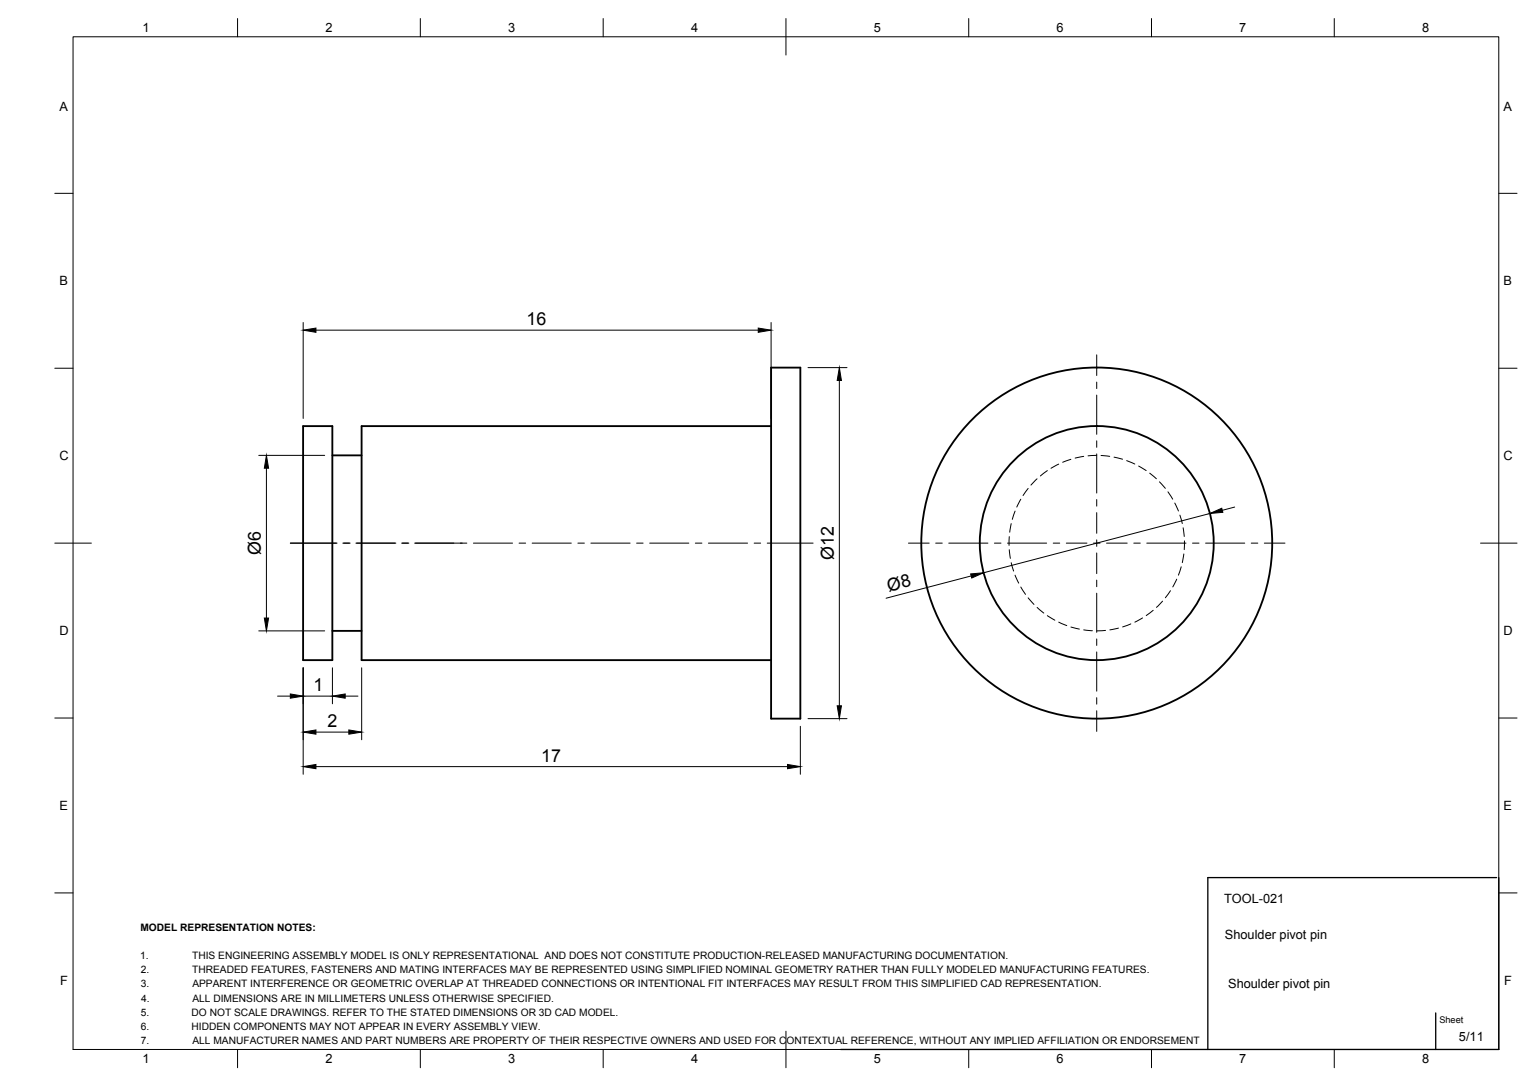
ISO-10303-21;
HEADER;
/* Generated by software containing ST-Developer
 * from STEP Tools, Inc. (www.steptools.com) 
 */

FILE_DESCRIPTION(
/* description */ (''),
/* implementation_level */ '2;1');

FILE_NAME(
/* name */ 'Shoulder pivot pin.step',
/* time_stamp */ '2026-11-10T09:05:57-08:00',
/* author */ (''),
/* organization */ (''),
/* preprocessor_version */ 'ST-DEVELOPER v20.2',
/* originating_system */ 'Autodesk Translation Framework v15.17.0.0',
/* authorisation */ '');

FILE_SCHEMA (('AUTOMOTIVE_DESIGN { 1 0 10303 214 3 1 1 }'));
ENDSEC;

DATA;
#10=MECHANICAL_DESIGN_GEOMETRIC_PRESENTATION_REPRESENTATION('',(#567),#19618);
#547=SHAPE_REPRESENTATION_RELATIONSHIP('SRR','None',#19666,#557);
#557=ADVANCED_BREP_SHAPE_REPRESENTATION('',(#577),#19609);
#567=STYLED_ITEM('',(#19729),#577);
#577=MANIFOLD_SOLID_BREP('Body1',#7105);
#605=FACE_BOUND('',#1304,.T.);
#606=FACE_BOUND('',#1306,.T.);
#607=FACE_BOUND('',#1309,.T.);
#698=PLANE('',#7347);
#699=PLANE('',#7349);
#700=PLANE('',#7353);
#701=PLANE('',#7358);
#702=PLANE('',#7360);
#883=FACE_OUTER_BOUND('',#1302,.T.);
#884=FACE_OUTER_BOUND('',#1303,.T.);
#885=FACE_OUTER_BOUND('',#1305,.T.);
#886=FACE_OUTER_BOUND('',#1307,.T.);
#887=FACE_OUTER_BOUND('',#1308,.T.);
#888=FACE_OUTER_BOUND('',#1310,.T.);
#889=FACE_OUTER_BOUND('',#1311,.T.);
#890=FACE_OUTER_BOUND('',#1312,.T.);
#891=FACE_OUTER_BOUND('',#1313,.T.);
#1302=EDGE_LOOP('',(#4842,#4843,#4844,#4845));
#1303=EDGE_LOOP('',(#4846));
#1304=EDGE_LOOP('',(#4847));
#1305=EDGE_LOOP('',(#4848));
#1306=EDGE_LOOP('',(#4849));
#1307=EDGE_LOOP('',(#4850,#4851,#4852,#4853));
#1308=EDGE_LOOP('',(#4854));
#1309=EDGE_LOOP('',(#4855));
#1310=EDGE_LOOP('',(#4856,#4857,#4858,#4859));
#1311=EDGE_LOOP('',(#4860));
#1312=EDGE_LOOP('',(#4861,#4862,#4863,#4864));
#1313=EDGE_LOOP('',(#4865));
#1813=LINE('',#9668,#2272);
#1814=LINE('',#9679,#2273);
#1815=LINE('',#9687,#2274);
#1816=LINE('',#9691,#2275);
#2272=VECTOR('',#8128,0.3);
#2273=VECTOR('',#8143,0.4);
#2274=VECTOR('',#8152,0.6);
#2275=VECTOR('',#8159,0.4);
#2670=CIRCLE('',#7345,0.3);
#2671=CIRCLE('',#7346,0.3);
#2672=CIRCLE('',#7348,0.4);
#2673=CIRCLE('',#7350,0.4);
#2674=CIRCLE('',#7352,0.4);
#2675=CIRCLE('',#7354,0.6);
#2676=CIRCLE('',#7355,0.4);
#2677=CIRCLE('',#7357,0.6);
#2921=VERTEX_POINT('',#9665);
#2922=VERTEX_POINT('',#9667);
#2923=VERTEX_POINT('',#9671);
#2924=VERTEX_POINT('',#9674);
#2925=VERTEX_POINT('',#9677);
#2926=VERTEX_POINT('',#9681);
#2927=VERTEX_POINT('',#9683);
#2928=VERTEX_POINT('',#9686);
#3646=EDGE_CURVE('',#2921,#2921,#2670,.T.);
#3647=EDGE_CURVE('',#2921,#2922,#1813,.T.);
#3648=EDGE_CURVE('',#2922,#2922,#2671,.T.);
#3649=EDGE_CURVE('',#2923,#2923,#2672,.T.);
#3650=EDGE_CURVE('',#2924,#2924,#2673,.T.);
#3651=EDGE_CURVE('',#2925,#2925,#2674,.T.);
#3652=EDGE_CURVE('',#2925,#2924,#1814,.T.);
#3653=EDGE_CURVE('',#2926,#2926,#2675,.T.);
#3654=EDGE_CURVE('',#2927,#2927,#2676,.T.);
#3655=EDGE_CURVE('',#2926,#2928,#1815,.T.);
#3656=EDGE_CURVE('',#2928,#2928,#2677,.T.);
#3657=EDGE_CURVE('',#2923,#2927,#1816,.T.);
#4842=ORIENTED_EDGE('',*,*,#3646,.T.);
#4843=ORIENTED_EDGE('',*,*,#3647,.T.);
#4844=ORIENTED_EDGE('',*,*,#3648,.F.);
#4845=ORIENTED_EDGE('',*,*,#3647,.F.);
#4846=ORIENTED_EDGE('',*,*,#3649,.F.);
#4847=ORIENTED_EDGE('',*,*,#3646,.F.);
#4848=ORIENTED_EDGE('',*,*,#3650,.F.);
#4849=ORIENTED_EDGE('',*,*,#3648,.T.);
#4850=ORIENTED_EDGE('',*,*,#3651,.F.);
#4851=ORIENTED_EDGE('',*,*,#3652,.T.);
#4852=ORIENTED_EDGE('',*,*,#3650,.T.);
#4853=ORIENTED_EDGE('',*,*,#3652,.F.);
#4854=ORIENTED_EDGE('',*,*,#3653,.T.);
#4855=ORIENTED_EDGE('',*,*,#3654,.F.);
#4856=ORIENTED_EDGE('',*,*,#3653,.F.);
#4857=ORIENTED_EDGE('',*,*,#3655,.T.);
#4858=ORIENTED_EDGE('',*,*,#3656,.T.);
#4859=ORIENTED_EDGE('',*,*,#3655,.F.);
#4860=ORIENTED_EDGE('',*,*,#3656,.F.);
#4861=ORIENTED_EDGE('',*,*,#3649,.T.);
#4862=ORIENTED_EDGE('',*,*,#3657,.T.);
#4863=ORIENTED_EDGE('',*,*,#3654,.T.);
#4864=ORIENTED_EDGE('',*,*,#3657,.F.);
#4865=ORIENTED_EDGE('',*,*,#3651,.T.);
#6579=CYLINDRICAL_SURFACE('',#7344,0.3);
#6580=CYLINDRICAL_SURFACE('',#7351,0.4);
#6581=CYLINDRICAL_SURFACE('',#7356,0.6);
#6582=CYLINDRICAL_SURFACE('',#7359,0.4);
#6762=ADVANCED_FACE('',(#883),#6579,.T.);
#6763=ADVANCED_FACE('',(#884,#605),#698,.F.);
#6764=ADVANCED_FACE('',(#885,#606),#699,.F.);
#6765=ADVANCED_FACE('',(#886),#6580,.T.);
#6766=ADVANCED_FACE('',(#887,#607),#700,.T.);
#6767=ADVANCED_FACE('',(#888),#6581,.T.);
#6768=ADVANCED_FACE('',(#889),#701,.F.);
#6769=ADVANCED_FACE('',(#890),#6582,.T.);
#6770=ADVANCED_FACE('',(#891),#702,.T.);
#7105=CLOSED_SHELL('',(#6762,#6763,#6764,#6765,#6766,#6767,#6768,#6769,
#6770));
#7343=AXIS2_PLACEMENT_3D('',#9663,#8122,#8123);
#7344=AXIS2_PLACEMENT_3D('',#9664,#8124,#8125);
#7345=AXIS2_PLACEMENT_3D('',#9666,#8126,#8127);
#7346=AXIS2_PLACEMENT_3D('',#9669,#8129,#8130);
#7347=AXIS2_PLACEMENT_3D('',#9670,#8131,#8132);
#7348=AXIS2_PLACEMENT_3D('',#9672,#8133,#8134);
#7349=AXIS2_PLACEMENT_3D('',#9673,#8135,#8136);
#7350=AXIS2_PLACEMENT_3D('',#9675,#8137,#8138);
#7351=AXIS2_PLACEMENT_3D('',#9676,#8139,#8140);
#7352=AXIS2_PLACEMENT_3D('',#9678,#8141,#8142);
#7353=AXIS2_PLACEMENT_3D('',#9680,#8144,#8145);
#7354=AXIS2_PLACEMENT_3D('',#9682,#8146,#8147);
#7355=AXIS2_PLACEMENT_3D('',#9684,#8148,#8149);
#7356=AXIS2_PLACEMENT_3D('',#9685,#8150,#8151);
#7357=AXIS2_PLACEMENT_3D('',#9688,#8153,#8154);
#7358=AXIS2_PLACEMENT_3D('',#9689,#8155,#8156);
#7359=AXIS2_PLACEMENT_3D('',#9690,#8157,#8158);
#7360=AXIS2_PLACEMENT_3D('',#9692,#8160,#8161);
#8122=DIRECTION('axis',(0.,0.,1.));
#8123=DIRECTION('refdir',(1.,0.,0.));
#8124=DIRECTION('center_axis',(0.,0.,1.));
#8125=DIRECTION('ref_axis',(1.,0.,0.));
#8126=DIRECTION('center_axis',(0.,0.,1.));
#8127=DIRECTION('ref_axis',(1.,0.,0.));
#8128=DIRECTION('',(0.,0.,1.));
#8129=DIRECTION('center_axis',(0.,0.,1.));
#8130=DIRECTION('ref_axis',(1.,0.,0.));
#8131=DIRECTION('center_axis',(0.,0.,-1.));
#8132=DIRECTION('ref_axis',(-1.,0.,0.));
#8133=DIRECTION('center_axis',(0.,0.,-1.));
#8134=DIRECTION('ref_axis',(1.,0.,0.));
#8135=DIRECTION('center_axis',(0.,0.,1.));
#8136=DIRECTION('ref_axis',(1.,0.,0.));
#8137=DIRECTION('center_axis',(0.,0.,1.));
#8138=DIRECTION('ref_axis',(1.,0.,0.));
#8139=DIRECTION('center_axis',(0.,0.,1.));
#8140=DIRECTION('ref_axis',(1.,0.,0.));
#8141=DIRECTION('center_axis',(0.,0.,1.));
#8142=DIRECTION('ref_axis',(1.,0.,0.));
#8143=DIRECTION('',(0.,0.,-1.));
#8144=DIRECTION('center_axis',(0.,0.,1.));
#8145=DIRECTION('ref_axis',(1.,0.,0.));
#8146=DIRECTION('center_axis',(0.,0.,1.));
#8147=DIRECTION('ref_axis',(1.,0.,0.));
#8148=DIRECTION('center_axis',(0.,0.,1.));
#8149=DIRECTION('ref_axis',(1.,0.,0.));
#8150=DIRECTION('center_axis',(0.,0.,1.));
#8151=DIRECTION('ref_axis',(1.,0.,0.));
#8152=DIRECTION('',(0.,0.,-1.));
#8153=DIRECTION('center_axis',(0.,0.,1.));
#8154=DIRECTION('ref_axis',(1.,0.,0.));
#8155=DIRECTION('center_axis',(0.,0.,1.));
#8156=DIRECTION('ref_axis',(1.,0.,0.));
#8157=DIRECTION('center_axis',(0.,0.,1.));
#8158=DIRECTION('ref_axis',(1.,0.,0.));
#8159=DIRECTION('',(0.,0.,-1.));
#8160=DIRECTION('center_axis',(0.,0.,1.));
#8161=DIRECTION('ref_axis',(1.,0.,0.));
#9663=CARTESIAN_POINT('',(0.,0.,0.));
#9664=CARTESIAN_POINT('Origin',(0.,0.,0.75));
#9665=CARTESIAN_POINT('',(-0.3,-3.67394039744206E-17,0.7));
#9666=CARTESIAN_POINT('Origin',(0.,0.,0.7));
#9667=CARTESIAN_POINT('',(-0.3,-3.67394039744206E-17,0.8));
#9668=CARTESIAN_POINT('',(-0.3,-3.67394039744206E-17,0.75));
#9669=CARTESIAN_POINT('Origin',(0.,0.,0.8));
#9670=CARTESIAN_POINT('Origin',(0.7,0.,0.7));
#9671=CARTESIAN_POINT('',(-0.4,4.89858719658941E-17,0.7));
#9672=CARTESIAN_POINT('Origin',(0.,0.,0.7));
#9673=CARTESIAN_POINT('Origin',(0.3,0.,0.8));
#9674=CARTESIAN_POINT('',(-0.4,-4.89858719658941E-17,0.8));
#9675=CARTESIAN_POINT('Origin',(0.,0.,0.8));
#9676=CARTESIAN_POINT('Origin',(0.,0.,-0.7));
#9677=CARTESIAN_POINT('',(-0.4,-4.89858719658941E-17,0.9));
#9678=CARTESIAN_POINT('Origin',(0.,0.,0.9));
#9679=CARTESIAN_POINT('',(-0.4,-4.89858719658941E-17,-0.7));
#9680=CARTESIAN_POINT('Origin',(0.,0.,-0.7));
#9681=CARTESIAN_POINT('',(-0.6,-7.34788079488412E-17,-0.7));
#9682=CARTESIAN_POINT('Origin',(0.,0.,-0.7));
#9683=CARTESIAN_POINT('',(-0.4,-4.89858719658941E-17,-0.7));
#9684=CARTESIAN_POINT('Origin',(0.,0.,-0.7));
#9685=CARTESIAN_POINT('Origin',(0.,0.,-0.8));
#9686=CARTESIAN_POINT('',(-0.6,-7.34788079488412E-17,-0.8));
#9687=CARTESIAN_POINT('',(-0.6,-7.34788079488412E-17,-0.8));
#9688=CARTESIAN_POINT('Origin',(0.,0.,-0.8));
#9689=CARTESIAN_POINT('Origin',(0.,0.,-0.8));
#9690=CARTESIAN_POINT('Origin',(0.,0.,-0.7));
#9691=CARTESIAN_POINT('',(-0.4,-4.89858719658941E-17,-0.7));
#9692=CARTESIAN_POINT('Origin',(0.,0.,0.9));
#19596=UNCERTAINTY_MEASURE_WITH_UNIT(LENGTH_MEASURE(0.001),#19619,
'DISTANCE_ACCURACY_VALUE',
'Maximum model space distance between geometric entities at asserted c
onnectivities');
#19605=UNCERTAINTY_MEASURE_WITH_UNIT(LENGTH_MEASURE(0.001),#19619,
'DISTANCE_ACCURACY_VALUE',
'Maximum model space distance between geometric entities at asserted c
onnectivities');
#19609=(
GEOMETRIC_REPRESENTATION_CONTEXT(3)
GLOBAL_UNCERTAINTY_ASSIGNED_CONTEXT((#19596))
GLOBAL_UNIT_ASSIGNED_CONTEXT((#19619,#19621,#19622))
REPRESENTATION_CONTEXT('','3D')
);
#19618=(
GEOMETRIC_REPRESENTATION_CONTEXT(3)
GLOBAL_UNCERTAINTY_ASSIGNED_CONTEXT((#19605))
GLOBAL_UNIT_ASSIGNED_CONTEXT((#19619,#19621,#19622))
REPRESENTATION_CONTEXT('','3D')
);
#19619=(
LENGTH_UNIT()
NAMED_UNIT(*)
SI_UNIT(.CENTI.,.METRE.)
);
#19621=(
NAMED_UNIT(*)
PLANE_ANGLE_UNIT()
SI_UNIT($,.RADIAN.)
);
#19622=(
NAMED_UNIT(*)
SI_UNIT($,.STERADIAN.)
SOLID_ANGLE_UNIT()
);
#19626=SHAPE_DEFINITION_REPRESENTATION(#19638,#19666);
#19638=PRODUCT_DEFINITION_SHAPE('',$,#19679);
#19666=SHAPE_REPRESENTATION('',(#7343),#19609);
#19675=PRODUCT_DEFINITION_CONTEXT('part definition',#19713,'design');
#19679=PRODUCT_DEFINITION('Shoulder pivot pin','Shoulder pivot pin',#19691,
#19675);
#19691=PRODUCT_DEFINITION_FORMATION('',$,#19718);
#19713=APPLICATION_CONTEXT(
'Core Data for Automotive Mechanical Design Process');
#19714=PRODUCT_CONTEXT('part definition',#19713,'mechanical');
#19718=PRODUCT('Shoulder pivot pin','Shoulder pivot pin',$,(#19714));
#19729=PRESENTATION_STYLE_ASSIGNMENT((#19737));
#19737=SURFACE_STYLE_USAGE(.BOTH.,#19745);
#19745=SURFACE_SIDE_STYLE('',(#19753));
#19753=SURFACE_STYLE_FILL_AREA(#19761);
#19761=FILL_AREA_STYLE('Pivot dark gray',(#19769));
#19769=FILL_AREA_STYLE_COLOUR('Pivot dark gray',#19777);
#19777=COLOUR_RGB('Pivot dark gray',0.27843137254902,0.309803921568627,
0.352941176470588);
ENDSEC;
END-ISO-10303-21;
